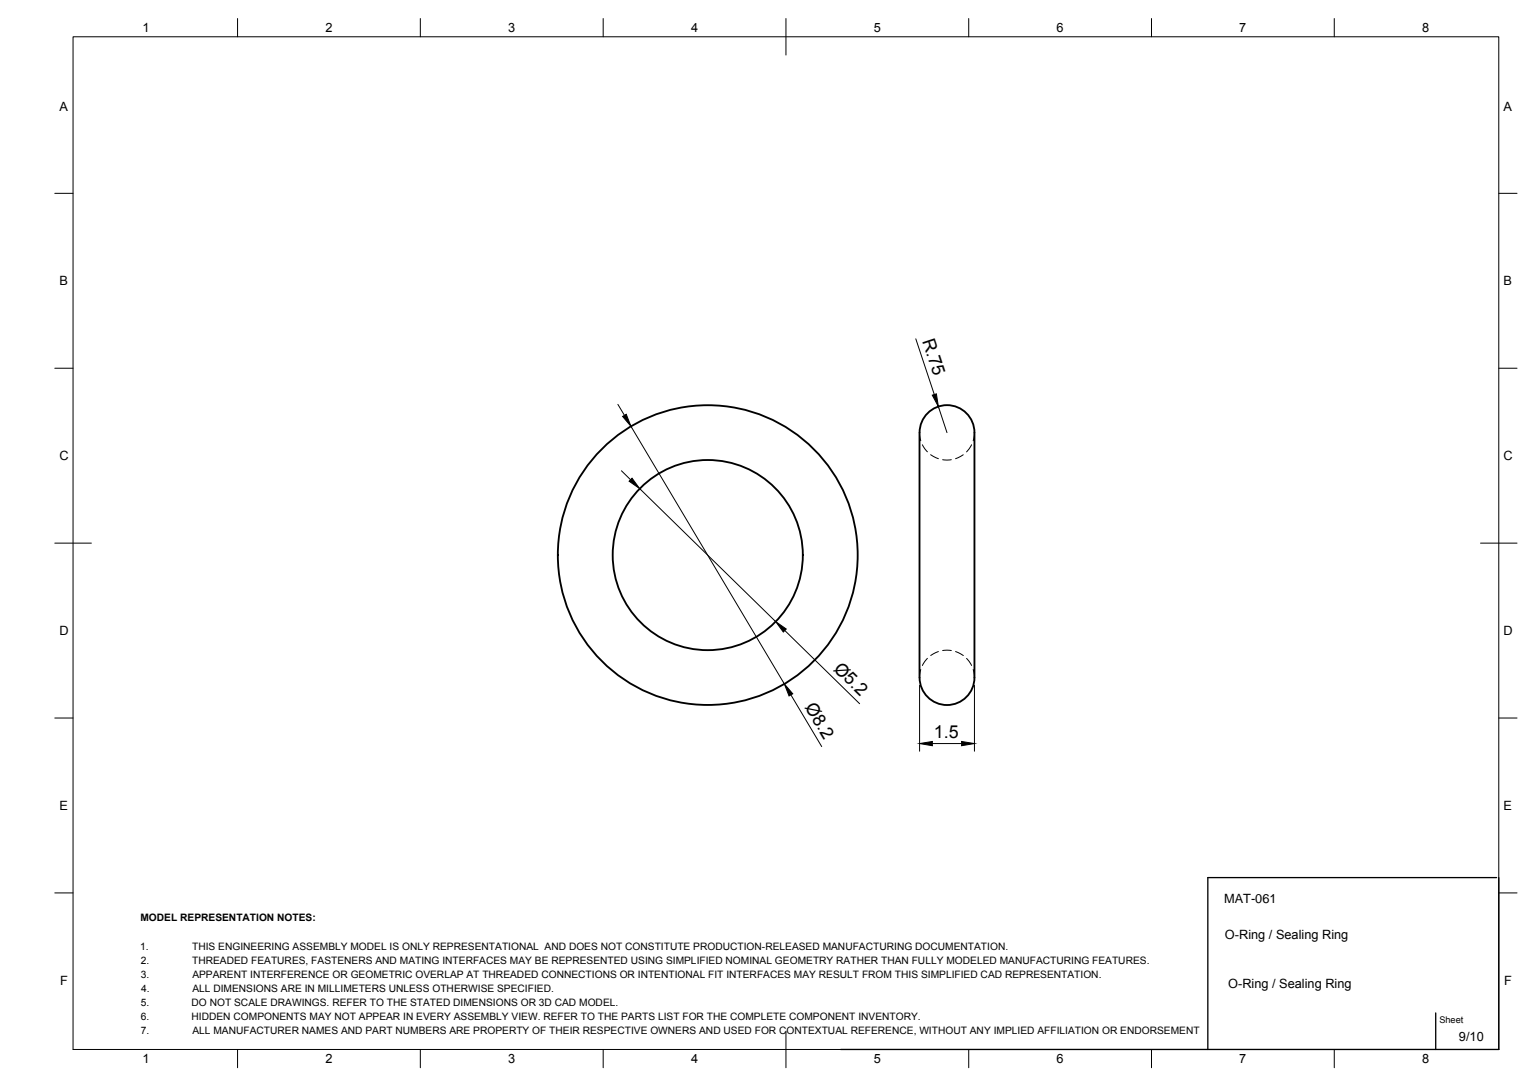
ISO-10303-21;
HEADER;
/* Generated by software containing ST-Developer
 * from STEP Tools, Inc. (www.steptools.com) 
 */

FILE_DESCRIPTION(
/* description */ ('', 'CAx-IF Rec.Pracs.---Representation and Presentation of Product Manufa
cturing Information (PMI)---4.0---2014-10-13'),
/* implementation_level */ '2;1');

FILE_NAME(
/* name */ 'O-Ring _ Sealing Ring.step',
/* time_stamp */ '2026-10-28T14:45:12+01:00',
/* author */ (''),
/* organization */ (''),
/* preprocessor_version */ 'ST-DEVELOPER v20.2',
/* originating_system */ 'Autodesk Translation Framework v15.17.0.0',
/* authorisation */ '');

FILE_SCHEMA (('AP242_MANAGED_MODEL_BASED_3D_ENGINEERING_MIM_LF { 1 0 10303 442 2 1 4 }'));
ENDSEC;

DATA;
#10=MECHANICAL_DESIGN_GEOMETRIC_PRESENTATION_REPRESENTATION('',(#268),#52164);
#231=TOROIDAL_SURFACE('',#10172,3.35,0.75);
#242=SHAPE_REPRESENTATION_RELATIONSHIP('SRR','None',#52221,#255);
#255=ADVANCED_BREP_SHAPE_REPRESENTATION('',(#281),#52161);
#268=STYLED_ITEM('',(#52325),#281);
#281=MANIFOLD_SOLID_BREP('Body1',#9128);
#1045=FACE_OUTER_BOUND('',#1614,.T.);
#1614=EDGE_LOOP('',(#8314,#8315,#8316,#8317));
#2081=CIRCLE('',#10173,0.75);
#2082=CIRCLE('',#10174,2.6);
#4244=VERTEX_POINT('',#52082);
#5603=EDGE_CURVE('',#4244,#4244,#2081,.T.);
#5604=EDGE_CURVE('',#4244,#4244,#2082,.T.);
#8314=ORIENTED_EDGE('',*,*,#5603,.F.);
#8315=ORIENTED_EDGE('',*,*,#5604,.T.);
#8316=ORIENTED_EDGE('',*,*,#5603,.T.);
#8317=ORIENTED_EDGE('',*,*,#5604,.F.);
#9108=ADVANCED_FACE('',(#1045),#231,.T.);
#9128=CLOSED_SHELL('',(#9108));
#10171=AXIS2_PLACEMENT_3D('',#52080,#12463,#12464);
#10172=AXIS2_PLACEMENT_3D('',#52081,#12465,#12466);
#10173=AXIS2_PLACEMENT_3D('',#52083,#12467,#12468);
#10174=AXIS2_PLACEMENT_3D('',#52084,#12469,#12470);
#12463=DIRECTION('axis',(0.,0.,1.));
#12464=DIRECTION('refdir',(1.,0.,0.));
#12465=DIRECTION('center_axis',(0.,0.,-1.));
#12466=DIRECTION('ref_axis',(1.,0.,0.));
#12467=DIRECTION('center_axis',(1.22464679914735E-16,1.,0.));
#12468=DIRECTION('ref_axis',(-1.,1.22464679914735E-16,0.));
#12469=DIRECTION('center_axis',(0.,0.,1.));
#12470=DIRECTION('ref_axis',(1.,0.,0.));
#52080=CARTESIAN_POINT('',(0.,0.,0.));
#52081=CARTESIAN_POINT('Origin',(0.,0.,-0.75));
#52082=CARTESIAN_POINT('',(-2.6,3.18408167778312E-16,-0.75));
#52083=CARTESIAN_POINT('Origin',(-3.35,4.10256677714363E-16,-0.75));
#52084=CARTESIAN_POINT('Origin',(0.,0.,-0.75));
#52146=UNCERTAINTY_MEASURE_WITH_UNIT(LENGTH_MEASURE(0.01),#52165,
'DISTANCE_ACCURACY_VALUE',
'Maximum model space distance between geometric entities at asserted c
onnectivities');
#52149=UNCERTAINTY_MEASURE_WITH_UNIT(LENGTH_MEASURE(0.01),#52165,
'DISTANCE_ACCURACY_VALUE',
'Maximum model space distance between geometric entities at asserted c
onnectivities');
#52161=(
GEOMETRIC_REPRESENTATION_CONTEXT(3)
GLOBAL_UNCERTAINTY_ASSIGNED_CONTEXT((#52146))
GLOBAL_UNIT_ASSIGNED_CONTEXT((#52165,#52167,#52168))
REPRESENTATION_CONTEXT('','3D')
);
#52164=(
GEOMETRIC_REPRESENTATION_CONTEXT(3)
GLOBAL_UNCERTAINTY_ASSIGNED_CONTEXT((#52149))
GLOBAL_UNIT_ASSIGNED_CONTEXT((#52165,#52167,#52168))
REPRESENTATION_CONTEXT('','3D')
);
#52165=(
LENGTH_UNIT()
NAMED_UNIT(*)
SI_UNIT(.MILLI.,.METRE.)
);
#52167=(
NAMED_UNIT(*)
PLANE_ANGLE_UNIT()
SI_UNIT($,.RADIAN.)
);
#52168=(
NAMED_UNIT(*)
SI_UNIT($,.STERADIAN.)
SOLID_ANGLE_UNIT()
);
#52180=SHAPE_DEFINITION_REPRESENTATION(#52194,#52221);
#52194=PRODUCT_DEFINITION_SHAPE('',$,#52236);
#52221=SHAPE_REPRESENTATION('',(#10171),#52161);
#52224=PRODUCT_DEFINITION_CONTEXT('part definition',#52268,'design');
#52236=PRODUCT_DEFINITION('O-Ring / Sealing Ring',
'O-Ring / Sealing Ring',#52250,#52224);
#52250=PRODUCT_DEFINITION_FORMATION('',$,#52281);
#52268=APPLICATION_CONTEXT('Managed model based 3d engineering');
#52269=PRODUCT_CONTEXT('part definition',#52268,'mechanical');
#52281=PRODUCT('O-Ring / Sealing Ring','O-Ring / Sealing Ring',
'NOT SPECIFIED',(#52269));
#52319=COLOUR_RGB('Black',0.12,0.14,0.17);
#52320=FILL_AREA_STYLE_COLOUR('',#52319);
#52321=FILL_AREA_STYLE('',(#52320));
#52322=SURFACE_STYLE_FILL_AREA(#52321);
#52323=SURFACE_SIDE_STYLE('',(#52322));
#52324=SURFACE_STYLE_USAGE(.BOTH.,#52323);
#52325=PRESENTATION_STYLE_ASSIGNMENT((#52324));
ENDSEC;
END-ISO-10303-21;
